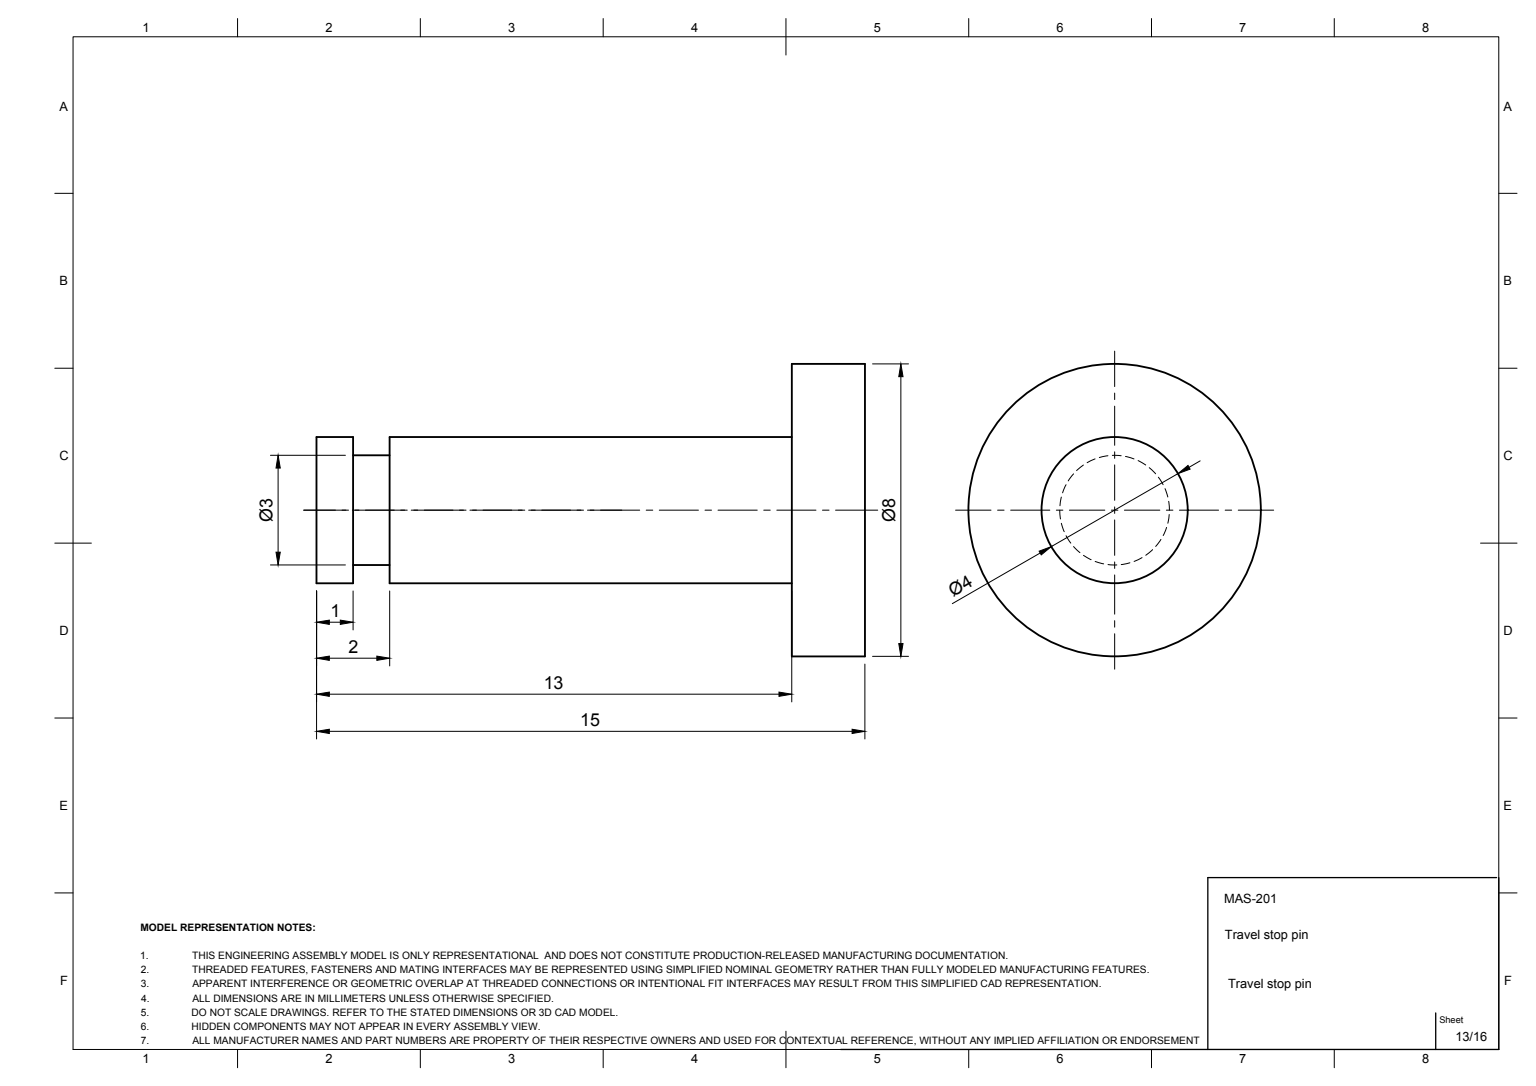
ISO-10303-21;
HEADER;
/* Generated by software containing ST-Developer
 * from STEP Tools, Inc. (www.steptools.com) 
 */

FILE_DESCRIPTION(
/* description */ ('Independent manual two-gate roller-track escapement for nominal30mm d
iameter20mm wide feed rollers. Opposed gates are driven by native capt
ured pin-slot loops with positive curved-slot travel stops at\X\B116de
g. Repeated gate/pin/washer/clip instances, adapted native common bear
ing families, full retaining lips and rotating polymer grip. External 
workpieces, gravity feeder/incline and mount anchors outside assembly.
 No powered-feed compatibility, impact, capacity, safety, force, wear 
or life rating.'),
/* implementation_level */ '2;1');

FILE_NAME(
/* name */ 'Travel stop pin.step',
/* time_stamp */ '2026-11-08T18:43:23-08:00',
/* author */ (''),
/* organization */ (''),
/* preprocessor_version */ 'ST-DEVELOPER v20.2',
/* originating_system */ 'Autodesk Translation Framework v15.17.0.0',
/* authorisation */ '');

FILE_SCHEMA (('AUTOMOTIVE_DESIGN { 1 0 10303 214 3 1 1 }'));
ENDSEC;

DATA;
#10=MECHANICAL_DESIGN_GEOMETRIC_PRESENTATION_REPRESENTATION('',(#467),#19863);
#429=SHAPE_REPRESENTATION_RELATIONSHIP('SRR','None',#19947,#448);
#448=ADVANCED_BREP_SHAPE_REPRESENTATION('',(#486),#19856);
#467=STYLED_ITEM('',(#20042),#486);
#486=MANIFOLD_SOLID_BREP('Body1',#6436);
#858=LINE('',#15947,#1323);
#859=LINE('',#15958,#1324);
#860=LINE('',#15966,#1325);
#861=LINE('',#15970,#1326);
#1323=VECTOR('',#8296,1.5);
#1324=VECTOR('',#8311,2.);
#1325=VECTOR('',#8320,4.);
#1326=VECTOR('',#8327,2.);
#1556=CYLINDRICAL_SURFACE('',#7021,1.5);
#1557=CYLINDRICAL_SURFACE('',#7028,2.);
#1558=CYLINDRICAL_SURFACE('',#7033,4.);
#1559=CYLINDRICAL_SURFACE('',#7036,2.);
#1673=FACE_BOUND('',#2360,.T.);
#1674=FACE_BOUND('',#2362,.T.);
#1675=FACE_BOUND('',#2365,.T.);
#1943=FACE_OUTER_BOUND('',#2358,.T.);
#1944=FACE_OUTER_BOUND('',#2359,.T.);
#1945=FACE_OUTER_BOUND('',#2361,.T.);
#1946=FACE_OUTER_BOUND('',#2363,.T.);
#1947=FACE_OUTER_BOUND('',#2364,.T.);
#1948=FACE_OUTER_BOUND('',#2366,.T.);
#1949=FACE_OUTER_BOUND('',#2367,.T.);
#1950=FACE_OUTER_BOUND('',#2368,.T.);
#1951=FACE_OUTER_BOUND('',#2369,.T.);
#2358=EDGE_LOOP('',(#5433,#5434,#5435,#5436));
#2359=EDGE_LOOP('',(#5437));
#2360=EDGE_LOOP('',(#5438));
#2361=EDGE_LOOP('',(#5439));
#2362=EDGE_LOOP('',(#5440));
#2363=EDGE_LOOP('',(#5441,#5442,#5443,#5444));
#2364=EDGE_LOOP('',(#5445));
#2365=EDGE_LOOP('',(#5446));
#2366=EDGE_LOOP('',(#5447,#5448,#5449,#5450));
#2367=EDGE_LOOP('',(#5451));
#2368=EDGE_LOOP('',(#5452,#5453,#5454,#5455));
#2369=EDGE_LOOP('',(#5456));
#2578=CIRCLE('',#7022,1.5);
#2579=CIRCLE('',#7023,1.5);
#2580=CIRCLE('',#7025,2.);
#2581=CIRCLE('',#7027,2.);
#2582=CIRCLE('',#7029,2.);
#2583=CIRCLE('',#7031,4.);
#2584=CIRCLE('',#7032,2.);
#2585=CIRCLE('',#7034,4.);
#3056=VERTEX_POINT('',#15944);
#3057=VERTEX_POINT('',#15946);
#3058=VERTEX_POINT('',#15950);
#3059=VERTEX_POINT('',#15953);
#3060=VERTEX_POINT('',#15956);
#3061=VERTEX_POINT('',#15960);
#3062=VERTEX_POINT('',#15962);
#3063=VERTEX_POINT('',#15965);
#3875=EDGE_CURVE('',#3056,#3056,#2578,.T.);
#3876=EDGE_CURVE('',#3056,#3057,#858,.T.);
#3877=EDGE_CURVE('',#3057,#3057,#2579,.T.);
#3878=EDGE_CURVE('',#3058,#3058,#2580,.T.);
#3879=EDGE_CURVE('',#3059,#3059,#2581,.T.);
#3880=EDGE_CURVE('',#3060,#3060,#2582,.T.);
#3881=EDGE_CURVE('',#3060,#3059,#859,.T.);
#3882=EDGE_CURVE('',#3061,#3061,#2583,.T.);
#3883=EDGE_CURVE('',#3062,#3062,#2584,.T.);
#3884=EDGE_CURVE('',#3061,#3063,#860,.T.);
#3885=EDGE_CURVE('',#3063,#3063,#2585,.T.);
#3886=EDGE_CURVE('',#3058,#3062,#861,.T.);
#5433=ORIENTED_EDGE('',*,*,#3875,.T.);
#5434=ORIENTED_EDGE('',*,*,#3876,.T.);
#5435=ORIENTED_EDGE('',*,*,#3877,.F.);
#5436=ORIENTED_EDGE('',*,*,#3876,.F.);
#5437=ORIENTED_EDGE('',*,*,#3878,.F.);
#5438=ORIENTED_EDGE('',*,*,#3875,.F.);
#5439=ORIENTED_EDGE('',*,*,#3879,.F.);
#5440=ORIENTED_EDGE('',*,*,#3877,.T.);
#5441=ORIENTED_EDGE('',*,*,#3880,.F.);
#5442=ORIENTED_EDGE('',*,*,#3881,.T.);
#5443=ORIENTED_EDGE('',*,*,#3879,.T.);
#5444=ORIENTED_EDGE('',*,*,#3881,.F.);
#5445=ORIENTED_EDGE('',*,*,#3882,.T.);
#5446=ORIENTED_EDGE('',*,*,#3883,.F.);
#5447=ORIENTED_EDGE('',*,*,#3882,.F.);
#5448=ORIENTED_EDGE('',*,*,#3884,.T.);
#5449=ORIENTED_EDGE('',*,*,#3885,.T.);
#5450=ORIENTED_EDGE('',*,*,#3884,.F.);
#5451=ORIENTED_EDGE('',*,*,#3885,.F.);
#5452=ORIENTED_EDGE('',*,*,#3878,.T.);
#5453=ORIENTED_EDGE('',*,*,#3886,.T.);
#5454=ORIENTED_EDGE('',*,*,#3883,.T.);
#5455=ORIENTED_EDGE('',*,*,#3886,.F.);
#5456=ORIENTED_EDGE('',*,*,#3880,.T.);
#6030=PLANE('',#7024);
#6031=PLANE('',#7026);
#6032=PLANE('',#7030);
#6033=PLANE('',#7035);
#6034=PLANE('',#7037);
#6322=ADVANCED_FACE('',(#1943),#1556,.T.);
#6323=ADVANCED_FACE('',(#1944,#1673),#6030,.F.);
#6324=ADVANCED_FACE('',(#1945,#1674),#6031,.F.);
#6325=ADVANCED_FACE('',(#1946),#1557,.T.);
#6326=ADVANCED_FACE('',(#1947,#1675),#6032,.T.);
#6327=ADVANCED_FACE('',(#1948),#1558,.T.);
#6328=ADVANCED_FACE('',(#1949),#6033,.F.);
#6329=ADVANCED_FACE('',(#1950),#1559,.T.);
#6330=ADVANCED_FACE('',(#1951),#6034,.T.);
#6436=CLOSED_SHELL('',(#6322,#6323,#6324,#6325,#6326,#6327,#6328,#6329,
#6330));
#7020=AXIS2_PLACEMENT_3D('',#15942,#8290,#8291);
#7021=AXIS2_PLACEMENT_3D('',#15943,#8292,#8293);
#7022=AXIS2_PLACEMENT_3D('',#15945,#8294,#8295);
#7023=AXIS2_PLACEMENT_3D('',#15948,#8297,#8298);
#7024=AXIS2_PLACEMENT_3D('',#15949,#8299,#8300);
#7025=AXIS2_PLACEMENT_3D('',#15951,#8301,#8302);
#7026=AXIS2_PLACEMENT_3D('',#15952,#8303,#8304);
#7027=AXIS2_PLACEMENT_3D('',#15954,#8305,#8306);
#7028=AXIS2_PLACEMENT_3D('',#15955,#8307,#8308);
#7029=AXIS2_PLACEMENT_3D('',#15957,#8309,#8310);
#7030=AXIS2_PLACEMENT_3D('',#15959,#8312,#8313);
#7031=AXIS2_PLACEMENT_3D('',#15961,#8314,#8315);
#7032=AXIS2_PLACEMENT_3D('',#15963,#8316,#8317);
#7033=AXIS2_PLACEMENT_3D('',#15964,#8318,#8319);
#7034=AXIS2_PLACEMENT_3D('',#15967,#8321,#8322);
#7035=AXIS2_PLACEMENT_3D('',#15968,#8323,#8324);
#7036=AXIS2_PLACEMENT_3D('',#15969,#8325,#8326);
#7037=AXIS2_PLACEMENT_3D('',#15971,#8328,#8329);
#8290=DIRECTION('axis',(0.,0.,1.));
#8291=DIRECTION('refdir',(1.,0.,0.));
#8292=DIRECTION('center_axis',(0.,0.,1.));
#8293=DIRECTION('ref_axis',(1.,0.,0.));
#8294=DIRECTION('center_axis',(0.,0.,1.));
#8295=DIRECTION('ref_axis',(1.,0.,0.));
#8296=DIRECTION('',(0.,0.,1.));
#8297=DIRECTION('center_axis',(0.,0.,1.));
#8298=DIRECTION('ref_axis',(1.,0.,0.));
#8299=DIRECTION('center_axis',(0.,0.,-1.));
#8300=DIRECTION('ref_axis',(-1.,0.,0.));
#8301=DIRECTION('center_axis',(0.,0.,-1.));
#8302=DIRECTION('ref_axis',(1.,0.,0.));
#8303=DIRECTION('center_axis',(0.,0.,1.));
#8304=DIRECTION('ref_axis',(1.,0.,0.));
#8305=DIRECTION('center_axis',(0.,0.,1.));
#8306=DIRECTION('ref_axis',(1.,0.,0.));
#8307=DIRECTION('center_axis',(0.,0.,1.));
#8308=DIRECTION('ref_axis',(1.,0.,0.));
#8309=DIRECTION('center_axis',(0.,0.,1.));
#8310=DIRECTION('ref_axis',(1.,0.,0.));
#8311=DIRECTION('',(0.,0.,-1.));
#8312=DIRECTION('center_axis',(0.,0.,1.));
#8313=DIRECTION('ref_axis',(1.,0.,0.));
#8314=DIRECTION('center_axis',(0.,0.,1.));
#8315=DIRECTION('ref_axis',(1.,0.,0.));
#8316=DIRECTION('center_axis',(0.,0.,1.));
#8317=DIRECTION('ref_axis',(1.,0.,0.));
#8318=DIRECTION('center_axis',(0.,0.,1.));
#8319=DIRECTION('ref_axis',(1.,0.,0.));
#8320=DIRECTION('',(0.,0.,-1.));
#8321=DIRECTION('center_axis',(0.,0.,1.));
#8322=DIRECTION('ref_axis',(1.,0.,0.));
#8323=DIRECTION('center_axis',(0.,0.,1.));
#8324=DIRECTION('ref_axis',(1.,0.,0.));
#8325=DIRECTION('center_axis',(0.,0.,1.));
#8326=DIRECTION('ref_axis',(1.,0.,0.));
#8327=DIRECTION('',(0.,0.,-1.));
#8328=DIRECTION('center_axis',(0.,0.,1.));
#8329=DIRECTION('ref_axis',(1.,0.,0.));
#15942=CARTESIAN_POINT('',(0.,0.,0.));
#15943=CARTESIAN_POINT('Origin',(0.,0.,11.5));
#15944=CARTESIAN_POINT('',(-1.5,-1.83697019872103E-16,11.));
#15945=CARTESIAN_POINT('Origin',(0.,0.,11.));
#15946=CARTESIAN_POINT('',(-1.5,-1.83697019872103E-16,12.));
#15947=CARTESIAN_POINT('',(-1.5,-1.83697019872103E-16,11.5));
#15948=CARTESIAN_POINT('Origin',(0.,0.,12.));
#15949=CARTESIAN_POINT('Origin',(5.5,0.,11.));
#15950=CARTESIAN_POINT('',(-2.,2.44929359829471E-16,11.));
#15951=CARTESIAN_POINT('Origin',(0.,0.,11.));
#15952=CARTESIAN_POINT('Origin',(1.5,0.,12.));
#15953=CARTESIAN_POINT('',(-2.,-2.44929359829471E-16,12.));
#15954=CARTESIAN_POINT('Origin',(0.,0.,12.));
#15955=CARTESIAN_POINT('Origin',(0.,0.,0.));
#15956=CARTESIAN_POINT('',(-2.,-2.44929359829471E-16,13.));
#15957=CARTESIAN_POINT('Origin',(0.,0.,13.));
#15958=CARTESIAN_POINT('',(-2.,-2.44929359829471E-16,0.));
#15959=CARTESIAN_POINT('Origin',(0.,0.,0.));
#15960=CARTESIAN_POINT('',(-4.,-4.89858719658941E-16,0.));
#15961=CARTESIAN_POINT('Origin',(0.,0.,0.));
#15962=CARTESIAN_POINT('',(-2.,-2.44929359829471E-16,0.));
#15963=CARTESIAN_POINT('Origin',(0.,0.,0.));
#15964=CARTESIAN_POINT('Origin',(0.,0.,-2.));
#15965=CARTESIAN_POINT('',(-4.,-4.89858719658941E-16,-2.));
#15966=CARTESIAN_POINT('',(-4.,-4.89858719658941E-16,-2.));
#15967=CARTESIAN_POINT('Origin',(0.,0.,-2.));
#15968=CARTESIAN_POINT('Origin',(0.,0.,-2.));
#15969=CARTESIAN_POINT('Origin',(0.,0.,0.));
#15970=CARTESIAN_POINT('',(-2.,-2.44929359829471E-16,0.));
#15971=CARTESIAN_POINT('Origin',(0.,0.,13.));
#19835=UNCERTAINTY_MEASURE_WITH_UNIT(LENGTH_MEASURE(0.01),#19864,
'DISTANCE_ACCURACY_VALUE',
'Maximum model space distance between geometric entities at asserted c
onnectivities');
#19842=UNCERTAINTY_MEASURE_WITH_UNIT(LENGTH_MEASURE(0.01),#19864,
'DISTANCE_ACCURACY_VALUE',
'Maximum model space distance between geometric entities at asserted c
onnectivities');
#19856=(
GEOMETRIC_REPRESENTATION_CONTEXT(3)
GLOBAL_UNCERTAINTY_ASSIGNED_CONTEXT((#19835))
GLOBAL_UNIT_ASSIGNED_CONTEXT((#19864,#19866,#19867))
REPRESENTATION_CONTEXT('','3D')
);
#19863=(
GEOMETRIC_REPRESENTATION_CONTEXT(3)
GLOBAL_UNCERTAINTY_ASSIGNED_CONTEXT((#19842))
GLOBAL_UNIT_ASSIGNED_CONTEXT((#19864,#19866,#19867))
REPRESENTATION_CONTEXT('','3D')
);
#19864=(
LENGTH_UNIT()
NAMED_UNIT(*)
SI_UNIT(.MILLI.,.METRE.)
);
#19866=(
NAMED_UNIT(*)
PLANE_ANGLE_UNIT()
SI_UNIT($,.RADIAN.)
);
#19867=(
NAMED_UNIT(*)
SI_UNIT($,.STERADIAN.)
SOLID_ANGLE_UNIT()
);
#19881=SHAPE_DEFINITION_REPRESENTATION(#19901,#19947);
#19901=PRODUCT_DEFINITION_SHAPE('',$,#19968);
#19947=SHAPE_REPRESENTATION('',(#7020),#19856);
#19954=PRODUCT_DEFINITION_CONTEXT('part definition',#20016,'design');
#19968=PRODUCT_DEFINITION('Travel stop pin','Travel stop pin',#19988,#19954);
#19988=PRODUCT_DEFINITION_FORMATION('',$,#20031);
#20016=APPLICATION_CONTEXT(
'Core Data for Automotive Mechanical Design Process');
#20017=PRODUCT_CONTEXT('part definition',#20016,'mechanical');
#20031=PRODUCT('Travel stop pin','Travel stop pin',$,(#20017));
#20042=PRESENTATION_STYLE_ASSIGNMENT((#20049));
#20049=SURFACE_STYLE_USAGE(.BOTH.,#20056);
#20056=SURFACE_SIDE_STYLE('',(#20063));
#20063=SURFACE_STYLE_FILL_AREA(#20070);
#20070=FILL_AREA_STYLE('Gray',(#20077));
#20077=FILL_AREA_STYLE_COLOUR('Gray',#20084);
#20084=COLOUR_RGB('Gray',0.407843137254902,0.447058823529412,0.498039215686275);
ENDSEC;
END-ISO-10303-21;
